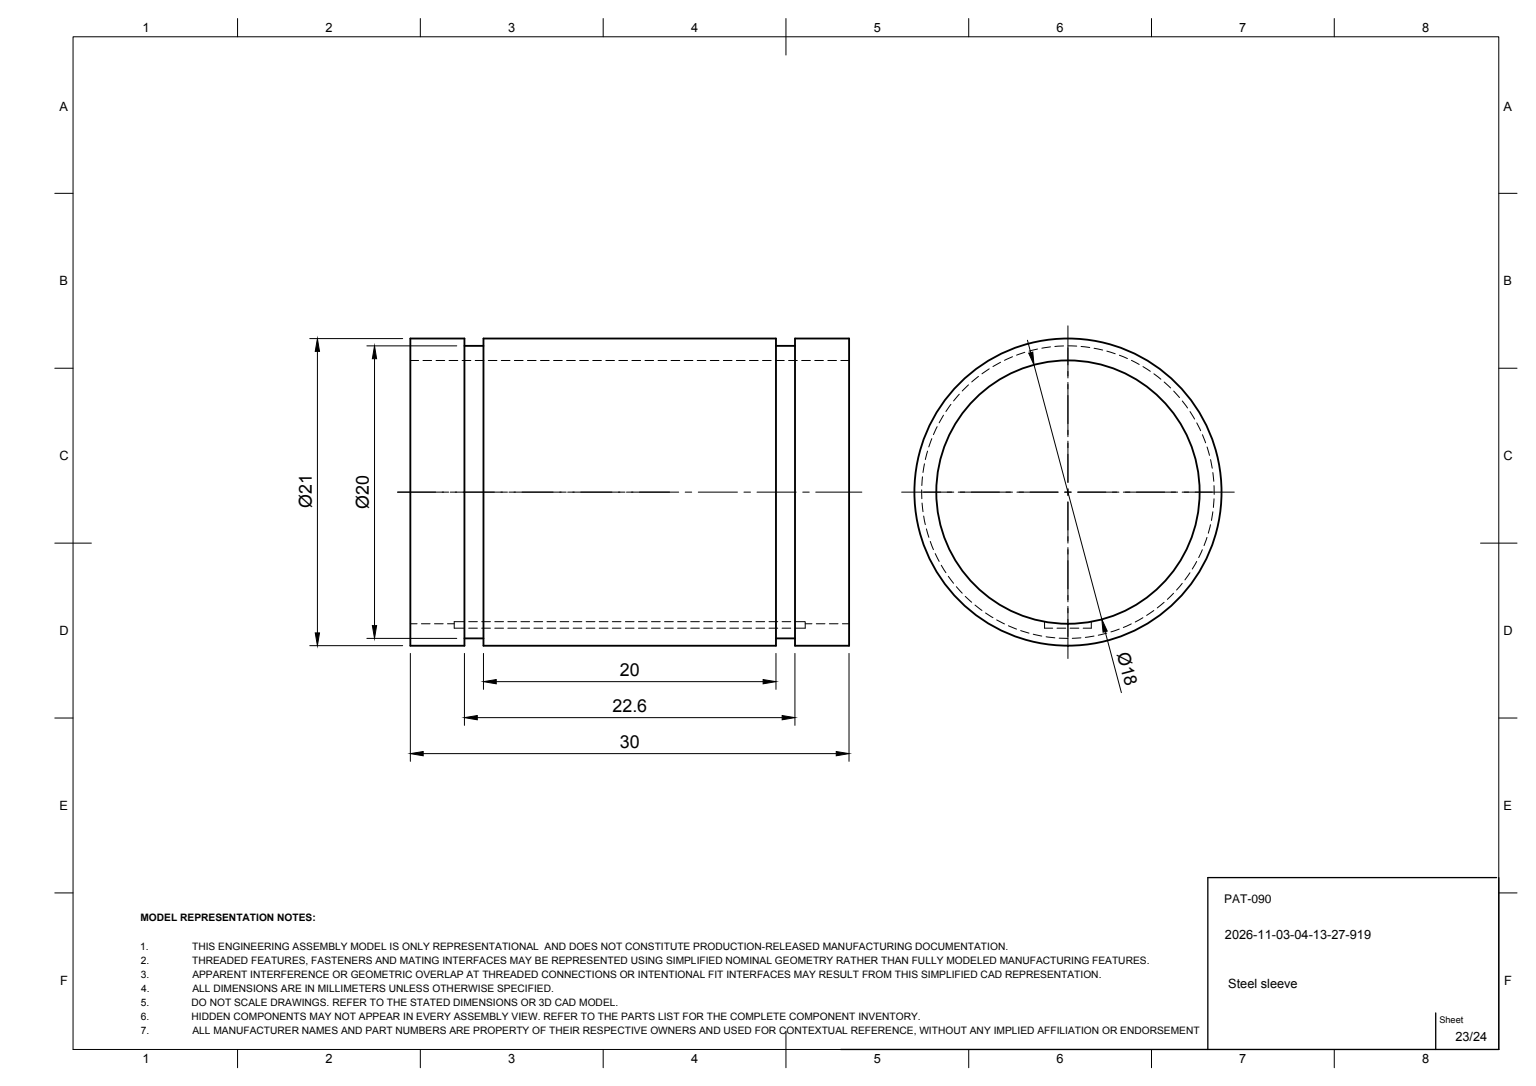
ISO-10303-21;
HEADER;
/* Generated by software containing ST-Developer
 * from STEP Tools, Inc. (www.steptools.com) 
 */

FILE_DESCRIPTION(
/* description */ ('Round-Shaft Linear Stage with Ball Bushings'),
/* implementation_level */ '2;1');

FILE_NAME(
/* name */ 'Steel sleeve.step',
/* time_stamp */ '2026-10-27T10:47:55-07:00',
/* author */ (''),
/* organization */ (''),
/* preprocessor_version */ 'ST-DEVELOPER v20.2',
/* originating_system */ 'Autodesk Translation Framework v15.17.0.0',
/* authorisation */ '');

FILE_SCHEMA (('AUTOMOTIVE_DESIGN { 1 0 10303 214 3 1 1 }'));
ENDSEC;

DATA;
#10=MECHANICAL_DESIGN_GEOMETRIC_PRESENTATION_REPRESENTATION('',(#317),#7835);
#275=SHAPE_REPRESENTATION_RELATIONSHIP('SRR','None',#7965,#296);
#296=ADVANCED_BREP_SHAPE_REPRESENTATION('',(#337),#7829);
#317=STYLED_ITEM('',(#8158),#337);
#337=MANIFOLD_SOLID_BREP('Body1',#4408);
#443=FACE_BOUND('',#1159,.T.);
#444=FACE_BOUND('',#1162,.T.);
#445=FACE_BOUND('',#1165,.T.);
#446=FACE_BOUND('',#1168,.T.);
#447=FACE_BOUND('',#1171,.T.);
#448=FACE_BOUND('',#1174,.T.);
#449=FACE_BOUND('',#1176,.T.);
#564=PLANE('',#4985);
#565=PLANE('',#4987);
#566=PLANE('',#4988);
#567=PLANE('',#4990);
#568=PLANE('',#4991);
#569=PLANE('',#4992);
#570=PLANE('',#4997);
#571=PLANE('',#5001);
#572=PLANE('',#5005);
#573=PLANE('',#5009);
#574=PLANE('',#5013);
#793=FACE_OUTER_BOUND('',#1153,.T.);
#794=FACE_OUTER_BOUND('',#1154,.T.);
#795=FACE_OUTER_BOUND('',#1155,.T.);
#796=FACE_OUTER_BOUND('',#1156,.T.);
#797=FACE_OUTER_BOUND('',#1157,.T.);
#798=FACE_OUTER_BOUND('',#1158,.T.);
#799=FACE_OUTER_BOUND('',#1160,.T.);
#800=FACE_OUTER_BOUND('',#1161,.T.);
#801=FACE_OUTER_BOUND('',#1163,.T.);
#802=FACE_OUTER_BOUND('',#1164,.T.);
#803=FACE_OUTER_BOUND('',#1166,.T.);
#804=FACE_OUTER_BOUND('',#1167,.T.);
#805=FACE_OUTER_BOUND('',#1169,.T.);
#806=FACE_OUTER_BOUND('',#1170,.T.);
#807=FACE_OUTER_BOUND('',#1172,.T.);
#808=FACE_OUTER_BOUND('',#1173,.T.);
#809=FACE_OUTER_BOUND('',#1175,.T.);
#1153=EDGE_LOOP('',(#3752,#3753,#3754,#3755));
#1154=EDGE_LOOP('',(#3756,#3757,#3758,#3759));
#1155=EDGE_LOOP('',(#3760,#3761,#3762,#3763));
#1156=EDGE_LOOP('',(#3764,#3765,#3766,#3767));
#1157=EDGE_LOOP('',(#3768,#3769,#3770,#3771));
#1158=EDGE_LOOP('',(#3772));
#1159=EDGE_LOOP('',(#3773));
#1160=EDGE_LOOP('',(#3774,#3775,#3776,#3777));
#1161=EDGE_LOOP('',(#3778));
#1162=EDGE_LOOP('',(#3779));
#1163=EDGE_LOOP('',(#3780,#3781,#3782,#3783));
#1164=EDGE_LOOP('',(#3784));
#1165=EDGE_LOOP('',(#3785));
#1166=EDGE_LOOP('',(#3786,#3787,#3788,#3789));
#1167=EDGE_LOOP('',(#3790));
#1168=EDGE_LOOP('',(#3791));
#1169=EDGE_LOOP('',(#3792,#3793,#3794,#3795));
#1170=EDGE_LOOP('',(#3796));
#1171=EDGE_LOOP('',(#3797));
#1172=EDGE_LOOP('',(#3798,#3799,#3800,#3801));
#1173=EDGE_LOOP('',(#3802));
#1174=EDGE_LOOP('',(#3803));
#1175=EDGE_LOOP('',(#3804,#3805,#3806,#3807));
#1176=EDGE_LOOP('',(#3808,#3809,#3810,#3811));
#1489=LINE('',#7402,#1829);
#1490=LINE('',#7404,#1830);
#1491=LINE('',#7405,#1831);
#1492=LINE('',#7408,#1832);
#1493=LINE('',#7410,#1833);
#1494=LINE('',#7411,#1834);
#1495=LINE('',#7416,#1835);
#1496=LINE('',#7417,#1836);
#1497=LINE('',#7419,#1837);
#1498=LINE('',#7420,#1838);
#1499=LINE('',#7430,#1839);
#1500=LINE('',#7437,#1840);
#1501=LINE('',#7444,#1841);
#1502=LINE('',#7451,#1842);
#1503=LINE('',#7458,#1843);
#1504=LINE('',#7463,#1844);
#1829=VECTOR('',#6092,1.);
#1830=VECTOR('',#6093,1.);
#1831=VECTOR('',#6094,1.);
#1832=VECTOR('',#6097,1.);
#1833=VECTOR('',#6098,1.);
#1834=VECTOR('',#6099,1.);
#1835=VECTOR('',#6104,1.);
#1836=VECTOR('',#6105,1.);
#1837=VECTOR('',#6108,1.);
#1838=VECTOR('',#6109,1.);
#1839=VECTOR('',#6122,1.05);
#1840=VECTOR('',#6131,1.);
#1841=VECTOR('',#6140,1.05);
#1842=VECTOR('',#6149,1.);
#1843=VECTOR('',#6158,1.05);
#1844=VECTOR('',#6165,0.9);
#2068=CIRCLE('',#4986,0.9);
#2069=CIRCLE('',#4989,0.9);
#2070=CIRCLE('',#4993,1.05);
#2071=CIRCLE('',#4994,0.9);
#2072=CIRCLE('',#4996,1.05);
#2073=CIRCLE('',#4998,1.);
#2074=CIRCLE('',#5000,1.);
#2075=CIRCLE('',#5002,1.05);
#2076=CIRCLE('',#5004,1.05);
#2077=CIRCLE('',#5006,1.);
#2078=CIRCLE('',#5008,1.);
#2079=CIRCLE('',#5010,1.05);
#2080=CIRCLE('',#5012,1.05);
#2081=CIRCLE('',#5014,0.9);
#2369=VERTEX_POINT('',#7398);
#2370=VERTEX_POINT('',#7399);
#2371=VERTEX_POINT('',#7401);
#2372=VERTEX_POINT('',#7403);
#2373=VERTEX_POINT('',#7407);
#2374=VERTEX_POINT('',#7409);
#2375=VERTEX_POINT('',#7413);
#2376=VERTEX_POINT('',#7415);
#2377=VERTEX_POINT('',#7423);
#2378=VERTEX_POINT('',#7425);
#2379=VERTEX_POINT('',#7428);
#2380=VERTEX_POINT('',#7432);
#2381=VERTEX_POINT('',#7435);
#2382=VERTEX_POINT('',#7439);
#2383=VERTEX_POINT('',#7442);
#2384=VERTEX_POINT('',#7446);
#2385=VERTEX_POINT('',#7449);
#2386=VERTEX_POINT('',#7453);
#2387=VERTEX_POINT('',#7456);
#2388=VERTEX_POINT('',#7460);
#2844=EDGE_CURVE('',#2369,#2370,#2068,.T.);
#2845=EDGE_CURVE('',#2371,#2369,#1489,.T.);
#2846=EDGE_CURVE('',#2372,#2371,#1490,.T.);
#2847=EDGE_CURVE('',#2370,#2372,#1491,.T.);
#2848=EDGE_CURVE('',#2370,#2373,#1492,.T.);
#2849=EDGE_CURVE('',#2374,#2372,#1493,.T.);
#2850=EDGE_CURVE('',#2374,#2373,#1494,.T.);
#2851=EDGE_CURVE('',#2373,#2375,#2069,.T.);
#2852=EDGE_CURVE('',#2376,#2374,#1495,.T.);
#2853=EDGE_CURVE('',#2375,#2376,#1496,.T.);
#2854=EDGE_CURVE('',#2375,#2369,#1497,.T.);
#2855=EDGE_CURVE('',#2376,#2371,#1498,.T.);
#2856=EDGE_CURVE('',#2377,#2377,#2070,.T.);
#2857=EDGE_CURVE('',#2378,#2378,#2071,.T.);
#2858=EDGE_CURVE('',#2379,#2379,#2072,.T.);
#2859=EDGE_CURVE('',#2379,#2377,#1499,.T.);
#2860=EDGE_CURVE('',#2380,#2380,#2073,.T.);
#2861=EDGE_CURVE('',#2381,#2381,#2074,.T.);
#2862=EDGE_CURVE('',#2381,#2380,#1500,.T.);
#2863=EDGE_CURVE('',#2382,#2382,#2075,.T.);
#2864=EDGE_CURVE('',#2383,#2383,#2076,.T.);
#2865=EDGE_CURVE('',#2383,#2382,#1501,.T.);
#2866=EDGE_CURVE('',#2384,#2384,#2077,.T.);
#2867=EDGE_CURVE('',#2385,#2385,#2078,.T.);
#2868=EDGE_CURVE('',#2385,#2384,#1502,.T.);
#2869=EDGE_CURVE('',#2386,#2386,#2079,.T.);
#2870=EDGE_CURVE('',#2387,#2387,#2080,.T.);
#2871=EDGE_CURVE('',#2387,#2386,#1503,.T.);
#2872=EDGE_CURVE('',#2388,#2388,#2081,.T.);
#2873=EDGE_CURVE('',#2388,#2378,#1504,.T.);
#3752=ORIENTED_EDGE('',*,*,#2844,.F.);
#3753=ORIENTED_EDGE('',*,*,#2845,.F.);
#3754=ORIENTED_EDGE('',*,*,#2846,.F.);
#3755=ORIENTED_EDGE('',*,*,#2847,.F.);
#3756=ORIENTED_EDGE('',*,*,#2848,.F.);
#3757=ORIENTED_EDGE('',*,*,#2847,.T.);
#3758=ORIENTED_EDGE('',*,*,#2849,.F.);
#3759=ORIENTED_EDGE('',*,*,#2850,.T.);
#3760=ORIENTED_EDGE('',*,*,#2851,.F.);
#3761=ORIENTED_EDGE('',*,*,#2850,.F.);
#3762=ORIENTED_EDGE('',*,*,#2852,.F.);
#3763=ORIENTED_EDGE('',*,*,#2853,.F.);
#3764=ORIENTED_EDGE('',*,*,#2854,.F.);
#3765=ORIENTED_EDGE('',*,*,#2853,.T.);
#3766=ORIENTED_EDGE('',*,*,#2855,.T.);
#3767=ORIENTED_EDGE('',*,*,#2845,.T.);
#3768=ORIENTED_EDGE('',*,*,#2855,.F.);
#3769=ORIENTED_EDGE('',*,*,#2852,.T.);
#3770=ORIENTED_EDGE('',*,*,#2849,.T.);
#3771=ORIENTED_EDGE('',*,*,#2846,.T.);
#3772=ORIENTED_EDGE('',*,*,#2856,.F.);
#3773=ORIENTED_EDGE('',*,*,#2857,.T.);
#3774=ORIENTED_EDGE('',*,*,#2858,.F.);
#3775=ORIENTED_EDGE('',*,*,#2859,.T.);
#3776=ORIENTED_EDGE('',*,*,#2856,.T.);
#3777=ORIENTED_EDGE('',*,*,#2859,.F.);
#3778=ORIENTED_EDGE('',*,*,#2858,.T.);
#3779=ORIENTED_EDGE('',*,*,#2860,.F.);
#3780=ORIENTED_EDGE('',*,*,#2861,.F.);
#3781=ORIENTED_EDGE('',*,*,#2862,.T.);
#3782=ORIENTED_EDGE('',*,*,#2860,.T.);
#3783=ORIENTED_EDGE('',*,*,#2862,.F.);
#3784=ORIENTED_EDGE('',*,*,#2863,.F.);
#3785=ORIENTED_EDGE('',*,*,#2861,.T.);
#3786=ORIENTED_EDGE('',*,*,#2864,.F.);
#3787=ORIENTED_EDGE('',*,*,#2865,.T.);
#3788=ORIENTED_EDGE('',*,*,#2863,.T.);
#3789=ORIENTED_EDGE('',*,*,#2865,.F.);
#3790=ORIENTED_EDGE('',*,*,#2864,.T.);
#3791=ORIENTED_EDGE('',*,*,#2866,.F.);
#3792=ORIENTED_EDGE('',*,*,#2867,.F.);
#3793=ORIENTED_EDGE('',*,*,#2868,.T.);
#3794=ORIENTED_EDGE('',*,*,#2866,.T.);
#3795=ORIENTED_EDGE('',*,*,#2868,.F.);
#3796=ORIENTED_EDGE('',*,*,#2869,.F.);
#3797=ORIENTED_EDGE('',*,*,#2867,.T.);
#3798=ORIENTED_EDGE('',*,*,#2870,.F.);
#3799=ORIENTED_EDGE('',*,*,#2871,.T.);
#3800=ORIENTED_EDGE('',*,*,#2869,.T.);
#3801=ORIENTED_EDGE('',*,*,#2871,.F.);
#3802=ORIENTED_EDGE('',*,*,#2870,.T.);
#3803=ORIENTED_EDGE('',*,*,#2872,.F.);
#3804=ORIENTED_EDGE('',*,*,#2872,.T.);
#3805=ORIENTED_EDGE('',*,*,#2873,.T.);
#3806=ORIENTED_EDGE('',*,*,#2857,.F.);
#3807=ORIENTED_EDGE('',*,*,#2873,.F.);
#3808=ORIENTED_EDGE('',*,*,#2851,.T.);
#3809=ORIENTED_EDGE('',*,*,#2854,.T.);
#3810=ORIENTED_EDGE('',*,*,#2844,.T.);
#3811=ORIENTED_EDGE('',*,*,#2848,.T.);
#4119=CYLINDRICAL_SURFACE('',#4995,1.05);
#4120=CYLINDRICAL_SURFACE('',#4999,1.);
#4121=CYLINDRICAL_SURFACE('',#5003,1.05);
#4122=CYLINDRICAL_SURFACE('',#5007,1.);
#4123=CYLINDRICAL_SURFACE('',#5011,1.05);
#4124=CYLINDRICAL_SURFACE('',#5015,0.9);
#4312=ADVANCED_FACE('',(#793),#564,.F.);
#4313=ADVANCED_FACE('',(#794),#565,.F.);
#4314=ADVANCED_FACE('',(#795),#566,.F.);
#4315=ADVANCED_FACE('',(#796),#567,.F.);
#4316=ADVANCED_FACE('',(#797),#568,.F.);
#4317=ADVANCED_FACE('',(#798,#443),#569,.T.);
#4318=ADVANCED_FACE('',(#799),#4119,.T.);
#4319=ADVANCED_FACE('',(#800,#444),#570,.T.);
#4320=ADVANCED_FACE('',(#801),#4120,.T.);
#4321=ADVANCED_FACE('',(#802,#445),#571,.T.);
#4322=ADVANCED_FACE('',(#803),#4121,.T.);
#4323=ADVANCED_FACE('',(#804,#446),#572,.T.);
#4324=ADVANCED_FACE('',(#805),#4122,.T.);
#4325=ADVANCED_FACE('',(#806,#447),#573,.T.);
#4326=ADVANCED_FACE('',(#807),#4123,.T.);
#4327=ADVANCED_FACE('',(#808,#448),#574,.T.);
#4328=ADVANCED_FACE('',(#809,#449),#4124,.F.);
#4408=CLOSED_SHELL('',(#4312,#4313,#4314,#4315,#4316,#4317,#4318,#4319,
#4320,#4321,#4322,#4323,#4324,#4325,#4326,#4327,#4328));
#4984=AXIS2_PLACEMENT_3D('',#7396,#6086,#6087);
#4985=AXIS2_PLACEMENT_3D('',#7397,#6088,#6089);
#4986=AXIS2_PLACEMENT_3D('',#7400,#6090,#6091);
#4987=AXIS2_PLACEMENT_3D('',#7406,#6095,#6096);
#4988=AXIS2_PLACEMENT_3D('',#7412,#6100,#6101);
#4989=AXIS2_PLACEMENT_3D('',#7414,#6102,#6103);
#4990=AXIS2_PLACEMENT_3D('',#7418,#6106,#6107);
#4991=AXIS2_PLACEMENT_3D('',#7421,#6110,#6111);
#4992=AXIS2_PLACEMENT_3D('',#7422,#6112,#6113);
#4993=AXIS2_PLACEMENT_3D('',#7424,#6114,#6115);
#4994=AXIS2_PLACEMENT_3D('',#7426,#6116,#6117);
#4995=AXIS2_PLACEMENT_3D('',#7427,#6118,#6119);
#4996=AXIS2_PLACEMENT_3D('',#7429,#6120,#6121);
#4997=AXIS2_PLACEMENT_3D('',#7431,#6123,#6124);
#4998=AXIS2_PLACEMENT_3D('',#7433,#6125,#6126);
#4999=AXIS2_PLACEMENT_3D('',#7434,#6127,#6128);
#5000=AXIS2_PLACEMENT_3D('',#7436,#6129,#6130);
#5001=AXIS2_PLACEMENT_3D('',#7438,#6132,#6133);
#5002=AXIS2_PLACEMENT_3D('',#7440,#6134,#6135);
#5003=AXIS2_PLACEMENT_3D('',#7441,#6136,#6137);
#5004=AXIS2_PLACEMENT_3D('',#7443,#6138,#6139);
#5005=AXIS2_PLACEMENT_3D('',#7445,#6141,#6142);
#5006=AXIS2_PLACEMENT_3D('',#7447,#6143,#6144);
#5007=AXIS2_PLACEMENT_3D('',#7448,#6145,#6146);
#5008=AXIS2_PLACEMENT_3D('',#7450,#6147,#6148);
#5009=AXIS2_PLACEMENT_3D('',#7452,#6150,#6151);
#5010=AXIS2_PLACEMENT_3D('',#7454,#6152,#6153);
#5011=AXIS2_PLACEMENT_3D('',#7455,#6154,#6155);
#5012=AXIS2_PLACEMENT_3D('',#7457,#6156,#6157);
#5013=AXIS2_PLACEMENT_3D('',#7459,#6159,#6160);
#5014=AXIS2_PLACEMENT_3D('',#7461,#6161,#6162);
#5015=AXIS2_PLACEMENT_3D('',#7462,#6163,#6164);
#6086=DIRECTION('axis',(0.,0.,1.));
#6087=DIRECTION('refdir',(1.,0.,0.));
#6088=DIRECTION('center_axis',(0.,1.,0.));
#6089=DIRECTION('ref_axis',(0.,0.,1.));
#6090=DIRECTION('center_axis',(0.,-1.,0.));
#6091=DIRECTION('ref_axis',(1.,0.,0.));
#6092=DIRECTION('',(-1.,0.,0.));
#6093=DIRECTION('',(0.,0.,-1.));
#6094=DIRECTION('',(1.,0.,0.));
#6095=DIRECTION('center_axis',(0.,0.,1.));
#6096=DIRECTION('ref_axis',(1.,0.,0.));
#6097=DIRECTION('',(0.,-1.,0.));
#6098=DIRECTION('',(0.,1.,0.));
#6099=DIRECTION('',(-1.,0.,0.));
#6100=DIRECTION('center_axis',(0.,-1.,0.));
#6101=DIRECTION('ref_axis',(0.,0.,-1.));
#6102=DIRECTION('center_axis',(0.,1.,0.));
#6103=DIRECTION('ref_axis',(1.,0.,0.));
#6104=DIRECTION('',(0.,0.,1.));
#6105=DIRECTION('',(1.,0.,0.));
#6106=DIRECTION('center_axis',(0.,0.,-1.));
#6107=DIRECTION('ref_axis',(-1.,0.,0.));
#6108=DIRECTION('',(0.,1.,0.));
#6109=DIRECTION('',(0.,1.,0.));
#6110=DIRECTION('center_axis',(1.,0.,0.));
#6111=DIRECTION('ref_axis',(0.,0.,-1.));
#6112=DIRECTION('center_axis',(0.,1.,0.));
#6113=DIRECTION('ref_axis',(0.,0.,1.));
#6114=DIRECTION('center_axis',(0.,-1.,0.));
#6115=DIRECTION('ref_axis',(1.,0.,0.));
#6116=DIRECTION('center_axis',(0.,-1.,0.));
#6117=DIRECTION('ref_axis',(1.,0.,0.));
#6118=DIRECTION('center_axis',(0.,-1.,0.));
#6119=DIRECTION('ref_axis',(1.,0.,0.));
#6120=DIRECTION('center_axis',(0.,-1.,0.));
#6121=DIRECTION('ref_axis',(1.,0.,0.));
#6122=DIRECTION('',(0.,1.,0.));
#6123=DIRECTION('center_axis',(0.,-1.,0.));
#6124=DIRECTION('ref_axis',(0.,0.,-1.));
#6125=DIRECTION('center_axis',(0.,-1.,0.));
#6126=DIRECTION('ref_axis',(1.,0.,0.));
#6127=DIRECTION('center_axis',(0.,-1.,0.));
#6128=DIRECTION('ref_axis',(1.,0.,0.));
#6129=DIRECTION('center_axis',(0.,-1.,0.));
#6130=DIRECTION('ref_axis',(1.,0.,0.));
#6131=DIRECTION('',(0.,1.,0.));
#6132=DIRECTION('center_axis',(0.,1.,0.));
#6133=DIRECTION('ref_axis',(0.,0.,1.));
#6134=DIRECTION('center_axis',(0.,-1.,0.));
#6135=DIRECTION('ref_axis',(1.,0.,0.));
#6136=DIRECTION('center_axis',(0.,-1.,0.));
#6137=DIRECTION('ref_axis',(1.,0.,0.));
#6138=DIRECTION('center_axis',(0.,-1.,0.));
#6139=DIRECTION('ref_axis',(1.,0.,0.));
#6140=DIRECTION('',(0.,1.,0.));
#6141=DIRECTION('center_axis',(0.,-1.,0.));
#6142=DIRECTION('ref_axis',(0.,0.,-1.));
#6143=DIRECTION('center_axis',(0.,-1.,0.));
#6144=DIRECTION('ref_axis',(1.,0.,0.));
#6145=DIRECTION('center_axis',(0.,-1.,0.));
#6146=DIRECTION('ref_axis',(1.,0.,0.));
#6147=DIRECTION('center_axis',(0.,-1.,0.));
#6148=DIRECTION('ref_axis',(1.,0.,0.));
#6149=DIRECTION('',(0.,1.,0.));
#6150=DIRECTION('center_axis',(0.,1.,0.));
#6151=DIRECTION('ref_axis',(0.,0.,1.));
#6152=DIRECTION('center_axis',(0.,-1.,0.));
#6153=DIRECTION('ref_axis',(1.,0.,0.));
#6154=DIRECTION('center_axis',(0.,-1.,0.));
#6155=DIRECTION('ref_axis',(1.,0.,0.));
#6156=DIRECTION('center_axis',(0.,-1.,0.));
#6157=DIRECTION('ref_axis',(1.,0.,0.));
#6158=DIRECTION('',(0.,1.,0.));
#6159=DIRECTION('center_axis',(0.,-1.,0.));
#6160=DIRECTION('ref_axis',(0.,0.,-1.));
#6161=DIRECTION('center_axis',(0.,-1.,0.));
#6162=DIRECTION('ref_axis',(1.,0.,0.));
#6163=DIRECTION('center_axis',(0.,-1.,0.));
#6164=DIRECTION('ref_axis',(1.,0.,0.));
#6165=DIRECTION('',(0.,1.,0.));
#7396=CARTESIAN_POINT('',(0.,0.,0.));
#7397=CARTESIAN_POINT('Origin',(0.75,1.2,0.));
#7398=CARTESIAN_POINT('',(0.885663593019381,1.2,-0.16));
#7399=CARTESIAN_POINT('',(0.885663593019381,1.2,0.16));
#7400=CARTESIAN_POINT('Origin',(0.,1.2,0.));
#7401=CARTESIAN_POINT('',(0.93,1.2,-0.16));
#7402=CARTESIAN_POINT('',(0.93,1.2,-0.16));
#7403=CARTESIAN_POINT('',(0.93,1.2,0.16));
#7404=CARTESIAN_POINT('',(0.93,1.2,0.16));
#7405=CARTESIAN_POINT('',(0.57,1.2,0.16));
#7406=CARTESIAN_POINT('Origin',(0.57,0.,0.16));
#7407=CARTESIAN_POINT('',(0.885663593019381,-1.2,0.16));
#7408=CARTESIAN_POINT('',(0.885663593019381,0.,0.16));
#7409=CARTESIAN_POINT('',(0.93,-1.2,0.16));
#7410=CARTESIAN_POINT('',(0.93,0.,0.16));
#7411=CARTESIAN_POINT('',(0.57,-1.2,0.16));
#7412=CARTESIAN_POINT('Origin',(0.75,-1.2,0.));
#7413=CARTESIAN_POINT('',(0.885663593019381,-1.2,-0.16));
#7414=CARTESIAN_POINT('Origin',(0.,-1.2,0.));
#7415=CARTESIAN_POINT('',(0.93,-1.2,-0.16));
#7416=CARTESIAN_POINT('',(0.93,-1.2,0.16));
#7417=CARTESIAN_POINT('',(0.93,-1.2,-0.16));
#7418=CARTESIAN_POINT('Origin',(0.93,0.,-0.16));
#7419=CARTESIAN_POINT('',(0.885663593019381,0.,-0.16));
#7420=CARTESIAN_POINT('',(0.93,0.,-0.16));
#7421=CARTESIAN_POINT('Origin',(0.93,0.,0.16));
#7422=CARTESIAN_POINT('Origin',(1.05,1.5,0.));
#7423=CARTESIAN_POINT('',(-1.05,1.5,-1.28587913910472E-16));
#7424=CARTESIAN_POINT('Origin',(0.,1.5,0.));
#7425=CARTESIAN_POINT('',(-0.9,1.5,-1.10218211923262E-16));
#7426=CARTESIAN_POINT('Origin',(0.,1.5,0.));
#7427=CARTESIAN_POINT('Origin',(0.,1.315,0.));
#7428=CARTESIAN_POINT('',(-1.05,1.13,-1.28587913910472E-16));
#7429=CARTESIAN_POINT('Origin',(0.,1.13,0.));
#7430=CARTESIAN_POINT('',(-1.05,1.315,-1.28587913910472E-16));
#7431=CARTESIAN_POINT('Origin',(1.,1.13,0.));
#7432=CARTESIAN_POINT('',(-1.,1.13,-1.22464679914735E-16));
#7433=CARTESIAN_POINT('Origin',(0.,1.13,0.));
#7434=CARTESIAN_POINT('Origin',(0.,1.065,0.));
#7435=CARTESIAN_POINT('',(-1.,1.,-1.22464679914735E-16));
#7436=CARTESIAN_POINT('Origin',(0.,1.,0.));
#7437=CARTESIAN_POINT('',(-1.,1.065,-1.22464679914735E-16));
#7438=CARTESIAN_POINT('Origin',(1.05,1.,0.));
#7439=CARTESIAN_POINT('',(-1.05,1.,-1.28587913910472E-16));
#7440=CARTESIAN_POINT('Origin',(0.,1.,0.));
#7441=CARTESIAN_POINT('Origin',(0.,0.,0.));
#7442=CARTESIAN_POINT('',(-1.05,-1.,-1.28587913910472E-16));
#7443=CARTESIAN_POINT('Origin',(0.,-1.,0.));
#7444=CARTESIAN_POINT('',(-1.05,0.,-1.28587913910472E-16));
#7445=CARTESIAN_POINT('Origin',(1.,-1.,0.));
#7446=CARTESIAN_POINT('',(-1.,-1.,-1.22464679914735E-16));
#7447=CARTESIAN_POINT('Origin',(0.,-1.,0.));
#7448=CARTESIAN_POINT('Origin',(0.,-1.065,0.));
#7449=CARTESIAN_POINT('',(-1.,-1.13,-1.22464679914735E-16));
#7450=CARTESIAN_POINT('Origin',(0.,-1.13,0.));
#7451=CARTESIAN_POINT('',(-1.,-1.065,-1.22464679914735E-16));
#7452=CARTESIAN_POINT('Origin',(1.05,-1.13,0.));
#7453=CARTESIAN_POINT('',(-1.05,-1.13,-1.28587913910472E-16));
#7454=CARTESIAN_POINT('Origin',(0.,-1.13,0.));
#7455=CARTESIAN_POINT('Origin',(0.,-1.315,0.));
#7456=CARTESIAN_POINT('',(-1.05,-1.5,-1.28587913910472E-16));
#7457=CARTESIAN_POINT('Origin',(0.,-1.5,0.));
#7458=CARTESIAN_POINT('',(-1.05,-1.315,-1.28587913910472E-16));
#7459=CARTESIAN_POINT('Origin',(0.9,-1.5,0.));
#7460=CARTESIAN_POINT('',(-0.9,-1.5,-1.10218211923262E-16));
#7461=CARTESIAN_POINT('Origin',(0.,-1.5,0.));
#7462=CARTESIAN_POINT('Origin',(0.,0.,0.));
#7463=CARTESIAN_POINT('',(-0.9,0.,-1.10218211923262E-16));
#7803=UNCERTAINTY_MEASURE_WITH_UNIT(LENGTH_MEASURE(0.001),#7836,
'DISTANCE_ACCURACY_VALUE',
'Maximum model space distance between geometric entities at asserted c
onnectivities');
#7809=UNCERTAINTY_MEASURE_WITH_UNIT(LENGTH_MEASURE(0.001),#7836,
'DISTANCE_ACCURACY_VALUE',
'Maximum model space distance between geometric entities at asserted c
onnectivities');
#7829=(
GEOMETRIC_REPRESENTATION_CONTEXT(3)
GLOBAL_UNCERTAINTY_ASSIGNED_CONTEXT((#7803))
GLOBAL_UNIT_ASSIGNED_CONTEXT((#7836,#7838,#7839))
REPRESENTATION_CONTEXT('','3D')
);
#7835=(
GEOMETRIC_REPRESENTATION_CONTEXT(3)
GLOBAL_UNCERTAINTY_ASSIGNED_CONTEXT((#7809))
GLOBAL_UNIT_ASSIGNED_CONTEXT((#7836,#7838,#7839))
REPRESENTATION_CONTEXT('','3D')
);
#7836=(
LENGTH_UNIT()
NAMED_UNIT(*)
SI_UNIT(.CENTI.,.METRE.)
);
#7838=(
NAMED_UNIT(*)
PLANE_ANGLE_UNIT()
SI_UNIT($,.RADIAN.)
);
#7839=(
NAMED_UNIT(*)
SI_UNIT($,.STERADIAN.)
SOLID_ANGLE_UNIT()
);
#7859=SHAPE_DEFINITION_REPRESENTATION(#7884,#7965);
#7884=PRODUCT_DEFINITION_SHAPE('',$,#7991);
#7965=SHAPE_REPRESENTATION('',(#4984),#7829);
#7971=PRODUCT_DEFINITION_CONTEXT('part definition',#8048,'design');
#7991=PRODUCT_DEFINITION('Steel sleeve','Steel sleeve',#8016,#7971);
#8016=PRODUCT_DEFINITION_FORMATION('',$,#8069);
#8048=APPLICATION_CONTEXT(
'Core Data for Automotive Mechanical Design Process');
#8049=PRODUCT_CONTEXT('part definition',#8048,'mechanical');
#8069=PRODUCT('Steel sleeve','Steel sleeve','Steel sleeve',(#8049));
#8152=COLOUR_RGB('Off White',0.89,0.88,0.83);
#8153=FILL_AREA_STYLE_COLOUR('',#8152);
#8154=FILL_AREA_STYLE('',(#8153));
#8155=SURFACE_STYLE_FILL_AREA(#8154);
#8156=SURFACE_SIDE_STYLE('',(#8155));
#8157=SURFACE_STYLE_USAGE(.BOTH.,#8156);
#8158=PRESENTATION_STYLE_ASSIGNMENT((#8157));
ENDSEC;
END-ISO-10303-21;
